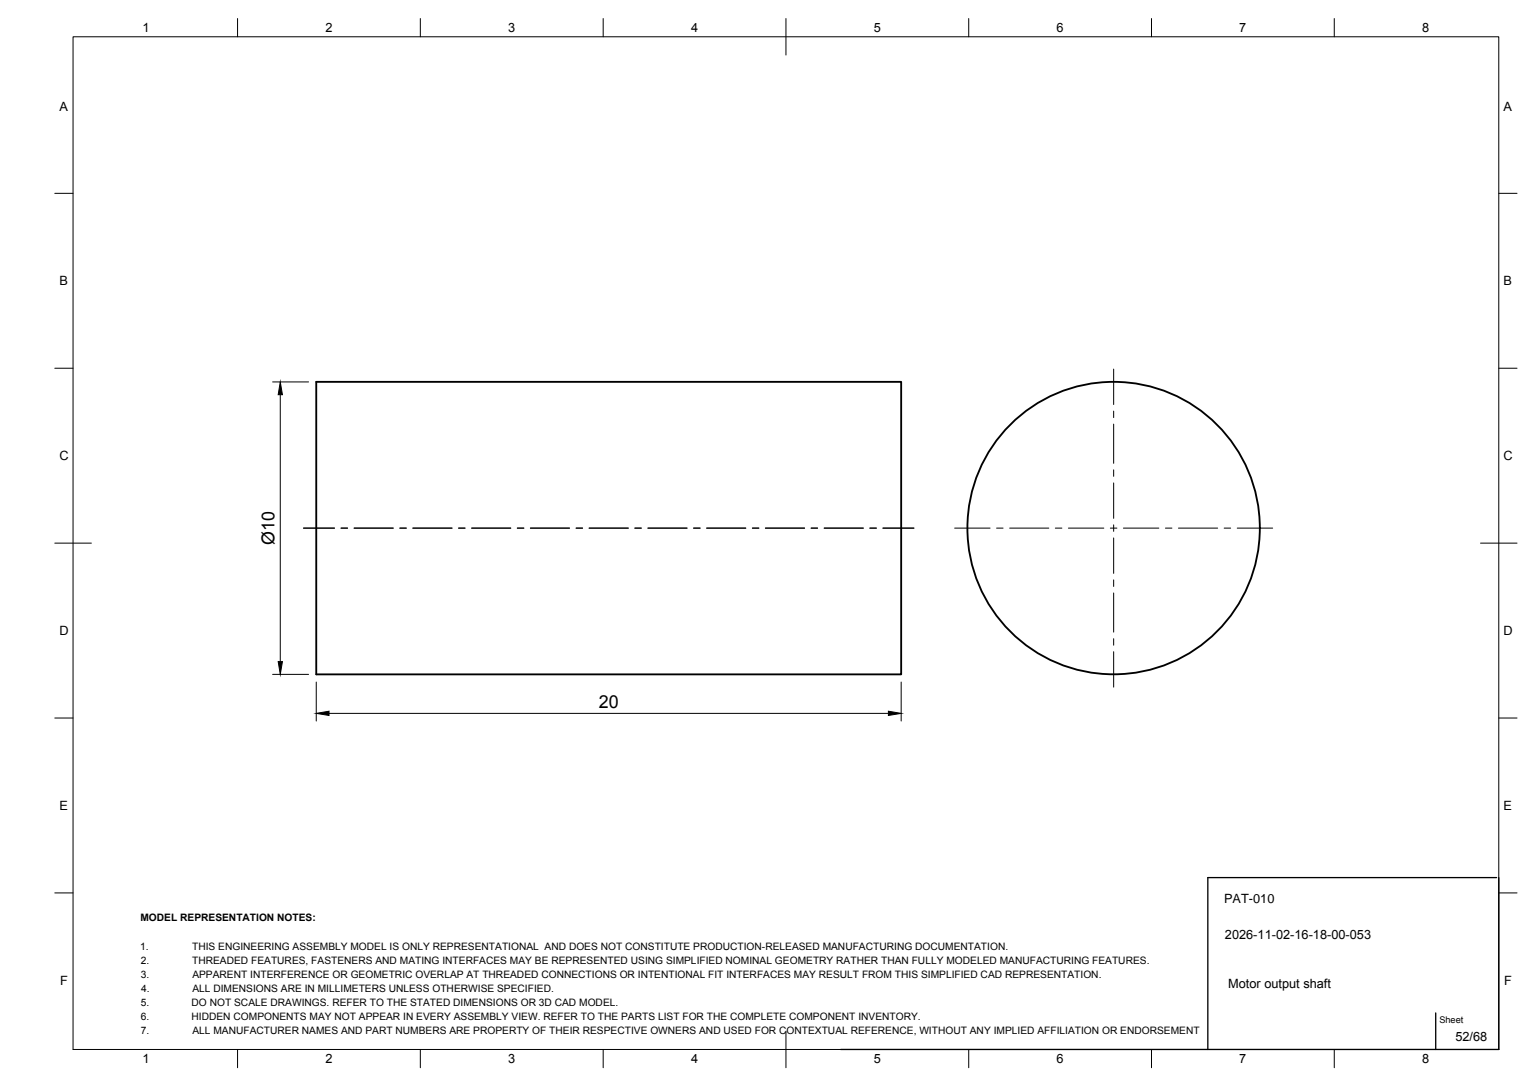
ISO-10303-21;
HEADER;
/* Generated by software containing ST-Developer
 * from STEP Tools, Inc. (www.steptools.com) 
 */

FILE_DESCRIPTION(
/* description */ ('Belt conveyor head drive unit'),
/* implementation_level */ '2;1');

FILE_NAME(
/* name */ 'Motor output shaft.step',
/* time_stamp */ '2026-10-28T03:26:19-07:00',
/* author */ (''),
/* organization */ (''),
/* preprocessor_version */ 'ST-DEVELOPER v20.2',
/* originating_system */ 'Autodesk Translation Framework v15.17.0.0',
/* authorisation */ '');

FILE_SCHEMA (('AUTOMOTIVE_DESIGN { 1 0 10303 214 3 1 1 }'));
ENDSEC;

DATA;
#10=MECHANICAL_DESIGN_GEOMETRIC_PRESENTATION_REPRESENTATION('',(#913),#27069);
#759=SHAPE_REPRESENTATION_RELATIONSHIP('SRR','None',#27407,#828);
#828=ADVANCED_BREP_SHAPE_REPRESENTATION('',(#994),#27049);
#913=STYLED_ITEM('',(#27797),#994);
#994=MANIFOLD_SOLID_BREP('Body1',#13782);
#1558=PLANE('',#15706);
#1559=PLANE('',#15707);
#2178=FACE_OUTER_BOUND('',#3182,.T.);
#2179=FACE_OUTER_BOUND('',#3183,.T.);
#2180=FACE_OUTER_BOUND('',#3184,.T.);
#3182=EDGE_LOOP('',(#11244,#11245,#11246,#11247));
#3183=EDGE_LOOP('',(#11248));
#3184=EDGE_LOOP('',(#11249));
#4058=LINE('',#24553,#4850);
#4850=VECTOR('',#19280,0.5);
#5609=CIRCLE('',#15704,0.5);
#5610=CIRCLE('',#15705,0.5);
#6735=VERTEX_POINT('',#24550);
#6736=VERTEX_POINT('',#24552);
#8314=EDGE_CURVE('',#6735,#6735,#5609,.T.);
#8315=EDGE_CURVE('',#6735,#6736,#4058,.T.);
#8316=EDGE_CURVE('',#6736,#6736,#5610,.T.);
#11244=ORIENTED_EDGE('',*,*,#8314,.F.);
#11245=ORIENTED_EDGE('',*,*,#8315,.T.);
#11246=ORIENTED_EDGE('',*,*,#8316,.T.);
#11247=ORIENTED_EDGE('',*,*,#8315,.F.);
#11248=ORIENTED_EDGE('',*,*,#8314,.T.);
#11249=ORIENTED_EDGE('',*,*,#8316,.F.);
#12738=CYLINDRICAL_SURFACE('',#15703,0.5);
#13457=ADVANCED_FACE('',(#2178),#12738,.T.);
#13458=ADVANCED_FACE('',(#2179),#1558,.T.);
#13459=ADVANCED_FACE('',(#2180),#1559,.F.);
#13782=CLOSED_SHELL('',(#13457,#13458,#13459));
#15702=AXIS2_PLACEMENT_3D('',#24548,#19274,#19275);
#15703=AXIS2_PLACEMENT_3D('',#24549,#19276,#19277);
#15704=AXIS2_PLACEMENT_3D('',#24551,#19278,#19279);
#15705=AXIS2_PLACEMENT_3D('',#24554,#19281,#19282);
#15706=AXIS2_PLACEMENT_3D('',#24555,#19283,#19284);
#15707=AXIS2_PLACEMENT_3D('',#24556,#19285,#19286);
#19274=DIRECTION('axis',(0.,0.,1.));
#19275=DIRECTION('refdir',(1.,0.,0.));
#19276=DIRECTION('center_axis',(0.,1.,0.));
#19277=DIRECTION('ref_axis',(1.,0.,0.));
#19278=DIRECTION('center_axis',(0.,1.,0.));
#19279=DIRECTION('ref_axis',(1.,0.,0.));
#19280=DIRECTION('',(0.,-1.,0.));
#19281=DIRECTION('center_axis',(0.,1.,0.));
#19282=DIRECTION('ref_axis',(1.,0.,0.));
#19283=DIRECTION('center_axis',(0.,1.,0.));
#19284=DIRECTION('ref_axis',(1.,0.,0.));
#19285=DIRECTION('center_axis',(0.,1.,0.));
#19286=DIRECTION('ref_axis',(1.,0.,0.));
#24548=CARTESIAN_POINT('',(0.,0.,0.));
#24549=CARTESIAN_POINT('Origin',(0.,3.,7.));
#24550=CARTESIAN_POINT('',(-0.5,5.,7.));
#24551=CARTESIAN_POINT('Origin',(0.,5.,7.));
#24552=CARTESIAN_POINT('',(-0.5,3.,7.));
#24553=CARTESIAN_POINT('',(-0.5,3.,7.));
#24554=CARTESIAN_POINT('Origin',(0.,3.,7.));
#24555=CARTESIAN_POINT('Origin',(0.,5.,7.));
#24556=CARTESIAN_POINT('Origin',(0.,3.,7.));
#26972=UNCERTAINTY_MEASURE_WITH_UNIT(LENGTH_MEASURE(0.001),#27070,
'DISTANCE_ACCURACY_VALUE',
'Maximum model space distance between geometric entities at asserted c
onnectivities');
#26992=UNCERTAINTY_MEASURE_WITH_UNIT(LENGTH_MEASURE(0.001),#27070,
'DISTANCE_ACCURACY_VALUE',
'Maximum model space distance between geometric entities at asserted c
onnectivities');
#27049=(
GEOMETRIC_REPRESENTATION_CONTEXT(3)
GLOBAL_UNCERTAINTY_ASSIGNED_CONTEXT((#26972))
GLOBAL_UNIT_ASSIGNED_CONTEXT((#27070,#27072,#27073))
REPRESENTATION_CONTEXT('','3D')
);
#27069=(
GEOMETRIC_REPRESENTATION_CONTEXT(3)
GLOBAL_UNCERTAINTY_ASSIGNED_CONTEXT((#26992))
GLOBAL_UNIT_ASSIGNED_CONTEXT((#27070,#27072,#27073))
REPRESENTATION_CONTEXT('','3D')
);
#27070=(
LENGTH_UNIT()
NAMED_UNIT(*)
SI_UNIT(.CENTI.,.METRE.)
);
#27072=(
NAMED_UNIT(*)
PLANE_ANGLE_UNIT()
SI_UNIT($,.RADIAN.)
);
#27073=(
NAMED_UNIT(*)
SI_UNIT($,.STERADIAN.)
SOLID_ANGLE_UNIT()
);
#27130=SHAPE_DEFINITION_REPRESENTATION(#27218,#27407);
#27218=PRODUCT_DEFINITION_SHAPE('',$,#27484);
#27407=SHAPE_REPRESENTATION('',(#15702),#27049);
#27427=PRODUCT_DEFINITION_CONTEXT('part definition',#27657,'design');
#27484=PRODUCT_DEFINITION('Motor output shaft','Motor output shaft',#27560,
#27427);
#27560=PRODUCT_DEFINITION_FORMATION('',$,#27715);
#27657=APPLICATION_CONTEXT(
'Core Data for Automotive Mechanical Design Process');
#27658=PRODUCT_CONTEXT('part definition',#27657,'mechanical');
#27715=PRODUCT('Motor output shaft','Motor output shaft',
'Motor output shaft',(#27658));
#27791=COLOUR_RGB('Grey',0.48,0.52,0.57);
#27792=FILL_AREA_STYLE_COLOUR('',#27791);
#27793=FILL_AREA_STYLE('',(#27792));
#27794=SURFACE_STYLE_FILL_AREA(#27793);
#27795=SURFACE_SIDE_STYLE('',(#27794));
#27796=SURFACE_STYLE_USAGE(.BOTH.,#27795);
#27797=PRESENTATION_STYLE_ASSIGNMENT((#27796));
ENDSEC;
END-ISO-10303-21;
